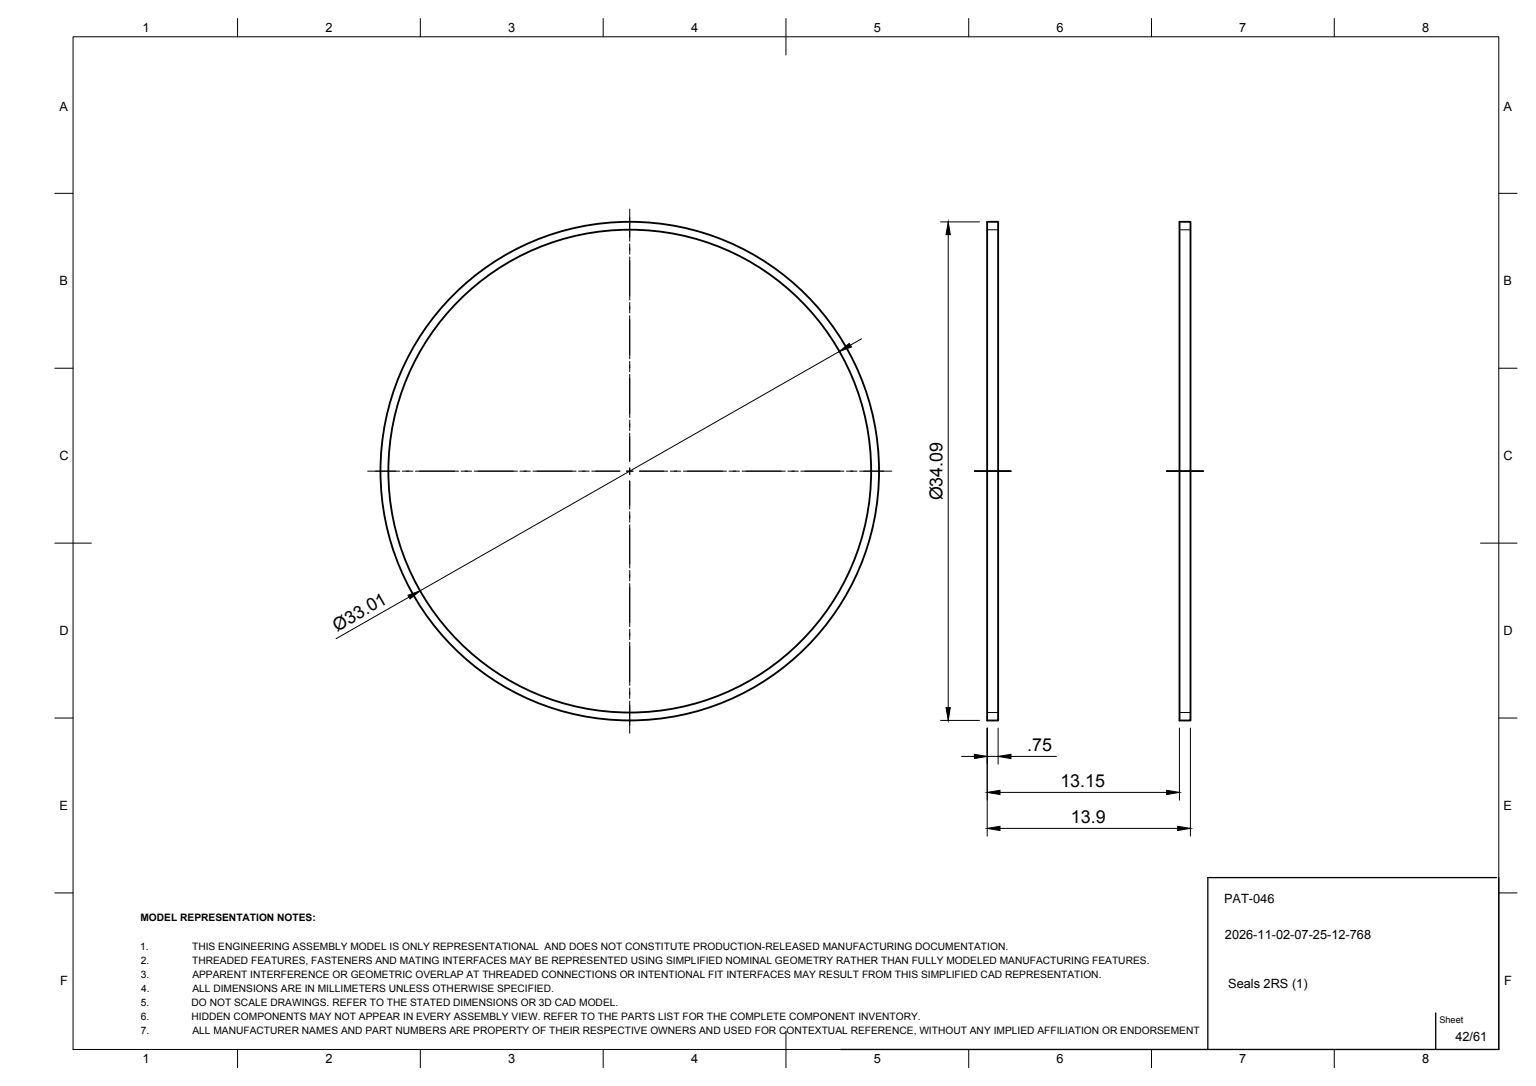
ISO-10303-21;
HEADER;
/* Generated by software containing ST-Developer
 * from STEP Tools, Inc. (www.steptools.com) 
 */

FILE_DESCRIPTION(
/* description */ ('Gear mesh backlash fixture'),
/* implementation_level */ '2;1');

FILE_NAME(
/* name */ 'Seals 2RS (1).step',
/* time_stamp */ '2026-10-28T03:26:00-07:00',
/* author */ (''),
/* organization */ (''),
/* preprocessor_version */ 'ST-DEVELOPER v20.2',
/* originating_system */ 'Autodesk Translation Framework v15.17.0.0',
/* authorisation */ '');

FILE_SCHEMA (('AUTOMOTIVE_DESIGN { 1 0 10303 214 3 1 1 }'));
ENDSEC;

DATA;
#10=MECHANICAL_DESIGN_GEOMETRIC_PRESENTATION_REPRESENTATION('',(#1062,#1063),#57900);
#948=SHAPE_REPRESENTATION_RELATIONSHIP('SRR','None',#58147,#998);
#998=ADVANCED_BREP_SHAPE_REPRESENTATION('',(#1125,#1126),#57880);
#1062=STYLED_ITEM('',(#58465),#1125);
#1063=STYLED_ITEM('',(#58465),#1126);
#1125=MANIFOLD_SOLID_BREP('Body1',#13624);
#1126=MANIFOLD_SOLID_BREP('Body2',#13625);
#1287=FACE_BOUND('',#2997,.T.);
#1288=FACE_BOUND('',#3000,.T.);
#1289=FACE_BOUND('',#3003,.T.);
#1290=FACE_BOUND('',#3006,.T.);
#1545=PLANE('',#15020);
#1546=PLANE('',#15025);
#1547=PLANE('',#15028);
#1548=PLANE('',#15033);
#2087=FACE_OUTER_BOUND('',#2996,.T.);
#2088=FACE_OUTER_BOUND('',#2998,.T.);
#2089=FACE_OUTER_BOUND('',#2999,.T.);
#2090=FACE_OUTER_BOUND('',#3001,.T.);
#2091=FACE_OUTER_BOUND('',#3002,.T.);
#2092=FACE_OUTER_BOUND('',#3004,.T.);
#2093=FACE_OUTER_BOUND('',#3005,.T.);
#2094=FACE_OUTER_BOUND('',#3007,.T.);
#2996=EDGE_LOOP('',(#10663));
#2997=EDGE_LOOP('',(#10664));
#2998=EDGE_LOOP('',(#10665,#10666,#10667,#10668));
#2999=EDGE_LOOP('',(#10669));
#3000=EDGE_LOOP('',(#10670));
#3001=EDGE_LOOP('',(#10671,#10672,#10673,#10674));
#3002=EDGE_LOOP('',(#10675));
#3003=EDGE_LOOP('',(#10676));
#3004=EDGE_LOOP('',(#10677,#10678,#10679,#10680));
#3005=EDGE_LOOP('',(#10681));
#3006=EDGE_LOOP('',(#10682));
#3007=EDGE_LOOP('',(#10683,#10684,#10685,#10686));
#3875=LINE('',#21973,#4764);
#3876=LINE('',#21978,#4765);
#3877=LINE('',#21987,#4766);
#3878=LINE('',#21992,#4767);
#4764=VECTOR('',#17702,1.70469);
#4765=VECTOR('',#17709,1.65031);
#4766=VECTOR('',#17720,1.70469);
#4767=VECTOR('',#17727,1.65031);
#5574=CIRCLE('',#15021,1.70469);
#5575=CIRCLE('',#15022,1.65031);
#5576=CIRCLE('',#15024,1.70469);
#5577=CIRCLE('',#15026,1.65031);
#5578=CIRCLE('',#15029,1.70469);
#5579=CIRCLE('',#15030,1.65031);
#5580=CIRCLE('',#15032,1.70469);
#5581=CIRCLE('',#15034,1.65031);
#6386=VERTEX_POINT('',#21966);
#6387=VERTEX_POINT('',#21968);
#6388=VERTEX_POINT('',#21971);
#6389=VERTEX_POINT('',#21975);
#6390=VERTEX_POINT('',#21980);
#6391=VERTEX_POINT('',#21982);
#6392=VERTEX_POINT('',#21985);
#6393=VERTEX_POINT('',#21989);
#7918=EDGE_CURVE('',#6386,#6386,#5574,.T.);
#7919=EDGE_CURVE('',#6387,#6387,#5575,.T.);
#7920=EDGE_CURVE('',#6388,#6388,#5576,.T.);
#7921=EDGE_CURVE('',#6388,#6386,#3875,.T.);
#7922=EDGE_CURVE('',#6389,#6389,#5577,.T.);
#7923=EDGE_CURVE('',#6389,#6387,#3876,.T.);
#7924=EDGE_CURVE('',#6390,#6390,#5578,.T.);
#7925=EDGE_CURVE('',#6391,#6391,#5579,.T.);
#7926=EDGE_CURVE('',#6392,#6392,#5580,.T.);
#7927=EDGE_CURVE('',#6392,#6390,#3877,.T.);
#7928=EDGE_CURVE('',#6393,#6393,#5581,.T.);
#7929=EDGE_CURVE('',#6393,#6391,#3878,.T.);
#10663=ORIENTED_EDGE('',*,*,#7918,.F.);
#10664=ORIENTED_EDGE('',*,*,#7919,.T.);
#10665=ORIENTED_EDGE('',*,*,#7920,.F.);
#10666=ORIENTED_EDGE('',*,*,#7921,.T.);
#10667=ORIENTED_EDGE('',*,*,#7918,.T.);
#10668=ORIENTED_EDGE('',*,*,#7921,.F.);
#10669=ORIENTED_EDGE('',*,*,#7920,.T.);
#10670=ORIENTED_EDGE('',*,*,#7922,.F.);
#10671=ORIENTED_EDGE('',*,*,#7922,.T.);
#10672=ORIENTED_EDGE('',*,*,#7923,.T.);
#10673=ORIENTED_EDGE('',*,*,#7919,.F.);
#10674=ORIENTED_EDGE('',*,*,#7923,.F.);
#10675=ORIENTED_EDGE('',*,*,#7924,.F.);
#10676=ORIENTED_EDGE('',*,*,#7925,.T.);
#10677=ORIENTED_EDGE('',*,*,#7926,.F.);
#10678=ORIENTED_EDGE('',*,*,#7927,.T.);
#10679=ORIENTED_EDGE('',*,*,#7924,.T.);
#10680=ORIENTED_EDGE('',*,*,#7927,.F.);
#10681=ORIENTED_EDGE('',*,*,#7926,.T.);
#10682=ORIENTED_EDGE('',*,*,#7928,.F.);
#10683=ORIENTED_EDGE('',*,*,#7928,.T.);
#10684=ORIENTED_EDGE('',*,*,#7929,.T.);
#10685=ORIENTED_EDGE('',*,*,#7925,.F.);
#10686=ORIENTED_EDGE('',*,*,#7929,.F.);
#12712=CYLINDRICAL_SURFACE('',#15023,1.70469);
#12713=CYLINDRICAL_SURFACE('',#15027,1.65031);
#12714=CYLINDRICAL_SURFACE('',#15031,1.70469);
#12715=CYLINDRICAL_SURFACE('',#15035,1.65031);
#13204=ADVANCED_FACE('',(#2087,#1287),#1545,.T.);
#13205=ADVANCED_FACE('',(#2088),#12712,.T.);
#13206=ADVANCED_FACE('',(#2089,#1288),#1546,.T.);
#13207=ADVANCED_FACE('',(#2090),#12713,.F.);
#13208=ADVANCED_FACE('',(#2091,#1289),#1547,.T.);
#13209=ADVANCED_FACE('',(#2092),#12714,.T.);
#13210=ADVANCED_FACE('',(#2093,#1290),#1548,.T.);
#13211=ADVANCED_FACE('',(#2094),#12715,.F.);
#13624=CLOSED_SHELL('',(#13204,#13205,#13206,#13207));
#13625=CLOSED_SHELL('',(#13208,#13209,#13210,#13211));
#15019=AXIS2_PLACEMENT_3D('',#21964,#17690,#17691);
#15020=AXIS2_PLACEMENT_3D('',#21965,#17692,#17693);
#15021=AXIS2_PLACEMENT_3D('',#21967,#17694,#17695);
#15022=AXIS2_PLACEMENT_3D('',#21969,#17696,#17697);
#15023=AXIS2_PLACEMENT_3D('',#21970,#17698,#17699);
#15024=AXIS2_PLACEMENT_3D('',#21972,#17700,#17701);
#15025=AXIS2_PLACEMENT_3D('',#21974,#17703,#17704);
#15026=AXIS2_PLACEMENT_3D('',#21976,#17705,#17706);
#15027=AXIS2_PLACEMENT_3D('',#21977,#17707,#17708);
#15028=AXIS2_PLACEMENT_3D('',#21979,#17710,#17711);
#15029=AXIS2_PLACEMENT_3D('',#21981,#17712,#17713);
#15030=AXIS2_PLACEMENT_3D('',#21983,#17714,#17715);
#15031=AXIS2_PLACEMENT_3D('',#21984,#17716,#17717);
#15032=AXIS2_PLACEMENT_3D('',#21986,#17718,#17719);
#15033=AXIS2_PLACEMENT_3D('',#21988,#17721,#17722);
#15034=AXIS2_PLACEMENT_3D('',#21990,#17723,#17724);
#15035=AXIS2_PLACEMENT_3D('',#21991,#17725,#17726);
#17690=DIRECTION('axis',(0.,0.,1.));
#17691=DIRECTION('refdir',(1.,0.,0.));
#17692=DIRECTION('center_axis',(0.,1.,0.));
#17693=DIRECTION('ref_axis',(0.,0.,1.));
#17694=DIRECTION('center_axis',(0.,-1.,0.));
#17695=DIRECTION('ref_axis',(1.,0.,0.));
#17696=DIRECTION('center_axis',(0.,-1.,0.));
#17697=DIRECTION('ref_axis',(1.,0.,0.));
#17698=DIRECTION('center_axis',(0.,-1.,0.));
#17699=DIRECTION('ref_axis',(1.,0.,0.));
#17700=DIRECTION('center_axis',(0.,-1.,0.));
#17701=DIRECTION('ref_axis',(1.,0.,0.));
#17702=DIRECTION('',(0.,1.,0.));
#17703=DIRECTION('center_axis',(0.,-1.,0.));
#17704=DIRECTION('ref_axis',(0.,0.,-1.));
#17705=DIRECTION('center_axis',(0.,-1.,0.));
#17706=DIRECTION('ref_axis',(1.,0.,0.));
#17707=DIRECTION('center_axis',(0.,-1.,0.));
#17708=DIRECTION('ref_axis',(1.,0.,0.));
#17709=DIRECTION('',(0.,1.,0.));
#17710=DIRECTION('center_axis',(0.,1.,0.));
#17711=DIRECTION('ref_axis',(0.,0.,1.));
#17712=DIRECTION('center_axis',(0.,-1.,0.));
#17713=DIRECTION('ref_axis',(1.,0.,0.));
#17714=DIRECTION('center_axis',(0.,-1.,0.));
#17715=DIRECTION('ref_axis',(1.,0.,0.));
#17716=DIRECTION('center_axis',(0.,-1.,0.));
#17717=DIRECTION('ref_axis',(1.,0.,0.));
#17718=DIRECTION('center_axis',(0.,-1.,0.));
#17719=DIRECTION('ref_axis',(1.,0.,0.));
#17720=DIRECTION('',(0.,1.,0.));
#17721=DIRECTION('center_axis',(0.,-1.,0.));
#17722=DIRECTION('ref_axis',(0.,0.,-1.));
#17723=DIRECTION('center_axis',(0.,-1.,0.));
#17724=DIRECTION('ref_axis',(1.,0.,0.));
#17725=DIRECTION('center_axis',(0.,-1.,0.));
#17726=DIRECTION('ref_axis',(1.,0.,0.));
#17727=DIRECTION('',(0.,1.,0.));
#21964=CARTESIAN_POINT('',(0.,0.,0.));
#21965=CARTESIAN_POINT('Origin',(1.70469,0.695,0.));
#21966=CARTESIAN_POINT('',(-1.70469,0.695,-2.0876431520385E-16));
#21967=CARTESIAN_POINT('Origin',(0.,0.695,0.));
#21968=CARTESIAN_POINT('',(-1.65031,0.695,-2.02104685910087E-16));
#21969=CARTESIAN_POINT('Origin',(0.,0.695,0.));
#21970=CARTESIAN_POINT('Origin',(0.,0.6575,0.));
#21971=CARTESIAN_POINT('',(-1.70469,0.62,-2.0876431520385E-16));
#21972=CARTESIAN_POINT('Origin',(0.,0.62,0.));
#21973=CARTESIAN_POINT('',(-1.70469,0.6575,-2.0876431520385E-16));
#21974=CARTESIAN_POINT('Origin',(1.65031,0.62,0.));
#21975=CARTESIAN_POINT('',(-1.65031,0.62,-2.02104685910087E-16));
#21976=CARTESIAN_POINT('Origin',(0.,0.62,0.));
#21977=CARTESIAN_POINT('Origin',(0.,0.6575,0.));
#21978=CARTESIAN_POINT('',(-1.65031,0.6575,-2.02104685910087E-16));
#21979=CARTESIAN_POINT('Origin',(1.70469,-0.62,0.));
#21980=CARTESIAN_POINT('',(-1.70469,-0.62,-2.0876431520385E-16));
#21981=CARTESIAN_POINT('Origin',(0.,-0.62,0.));
#21982=CARTESIAN_POINT('',(-1.65031,-0.62,-2.02104685910087E-16));
#21983=CARTESIAN_POINT('Origin',(0.,-0.62,0.));
#21984=CARTESIAN_POINT('Origin',(0.,-0.6575,0.));
#21985=CARTESIAN_POINT('',(-1.70469,-0.695,-2.0876431520385E-16));
#21986=CARTESIAN_POINT('Origin',(0.,-0.695,0.));
#21987=CARTESIAN_POINT('',(-1.70469,-0.6575,-2.0876431520385E-16));
#21988=CARTESIAN_POINT('Origin',(1.65031,-0.695,0.));
#21989=CARTESIAN_POINT('',(-1.65031,-0.695,-2.02104685910087E-16));
#21990=CARTESIAN_POINT('Origin',(0.,-0.695,0.));
#21991=CARTESIAN_POINT('Origin',(0.,-0.6575,0.));
#21992=CARTESIAN_POINT('',(-1.65031,-0.6575,-2.02104685910087E-16));
#57821=UNCERTAINTY_MEASURE_WITH_UNIT(LENGTH_MEASURE(0.001),#57901,
'DISTANCE_ACCURACY_VALUE',
'Maximum model space distance between geometric entities at asserted c
onnectivities');
#57841=UNCERTAINTY_MEASURE_WITH_UNIT(LENGTH_MEASURE(0.001),#57901,
'DISTANCE_ACCURACY_VALUE',
'Maximum model space distance between geometric entities at asserted c
onnectivities');
#57880=(
GEOMETRIC_REPRESENTATION_CONTEXT(3)
GLOBAL_UNCERTAINTY_ASSIGNED_CONTEXT((#57821))
GLOBAL_UNIT_ASSIGNED_CONTEXT((#57901,#57903,#57904))
REPRESENTATION_CONTEXT('','3D')
);
#57900=(
GEOMETRIC_REPRESENTATION_CONTEXT(3)
GLOBAL_UNCERTAINTY_ASSIGNED_CONTEXT((#57841))
GLOBAL_UNIT_ASSIGNED_CONTEXT((#57901,#57903,#57904))
REPRESENTATION_CONTEXT('','3D')
);
#57901=(
LENGTH_UNIT()
NAMED_UNIT(*)
SI_UNIT(.CENTI.,.METRE.)
);
#57903=(
NAMED_UNIT(*)
PLANE_ANGLE_UNIT()
SI_UNIT($,.RADIAN.)
);
#57904=(
NAMED_UNIT(*)
SI_UNIT($,.STERADIAN.)
SOLID_ANGLE_UNIT()
);
#57943=SHAPE_DEFINITION_REPRESENTATION(#58009,#58147);
#58009=PRODUCT_DEFINITION_SHAPE('',$,#58206);
#58147=SHAPE_REPRESENTATION('',(#15019),#57880);
#58167=PRODUCT_DEFINITION_CONTEXT('part definition',#58343,'design');
#58206=PRODUCT_DEFINITION('Seals 2RS (1)','Seals 2RS (1)',#58264,#58167);
#58264=PRODUCT_DEFINITION_FORMATION('',$,#58383);
#58343=APPLICATION_CONTEXT(
'Core Data for Automotive Mechanical Design Process');
#58344=PRODUCT_CONTEXT('part definition',#58343,'mechanical');
#58383=PRODUCT('Seals 2RS (1)','Seals 2RS (1)','Seals 2RS (1)',(#58344));
#58459=COLOUR_RGB('Grey',0.48,0.52,0.57);
#58460=FILL_AREA_STYLE_COLOUR('',#58459);
#58461=FILL_AREA_STYLE('',(#58460));
#58462=SURFACE_STYLE_FILL_AREA(#58461);
#58463=SURFACE_SIDE_STYLE('',(#58462));
#58464=SURFACE_STYLE_USAGE(.BOTH.,#58463);
#58465=PRESENTATION_STYLE_ASSIGNMENT((#58464));
ENDSEC;
END-ISO-10303-21;
